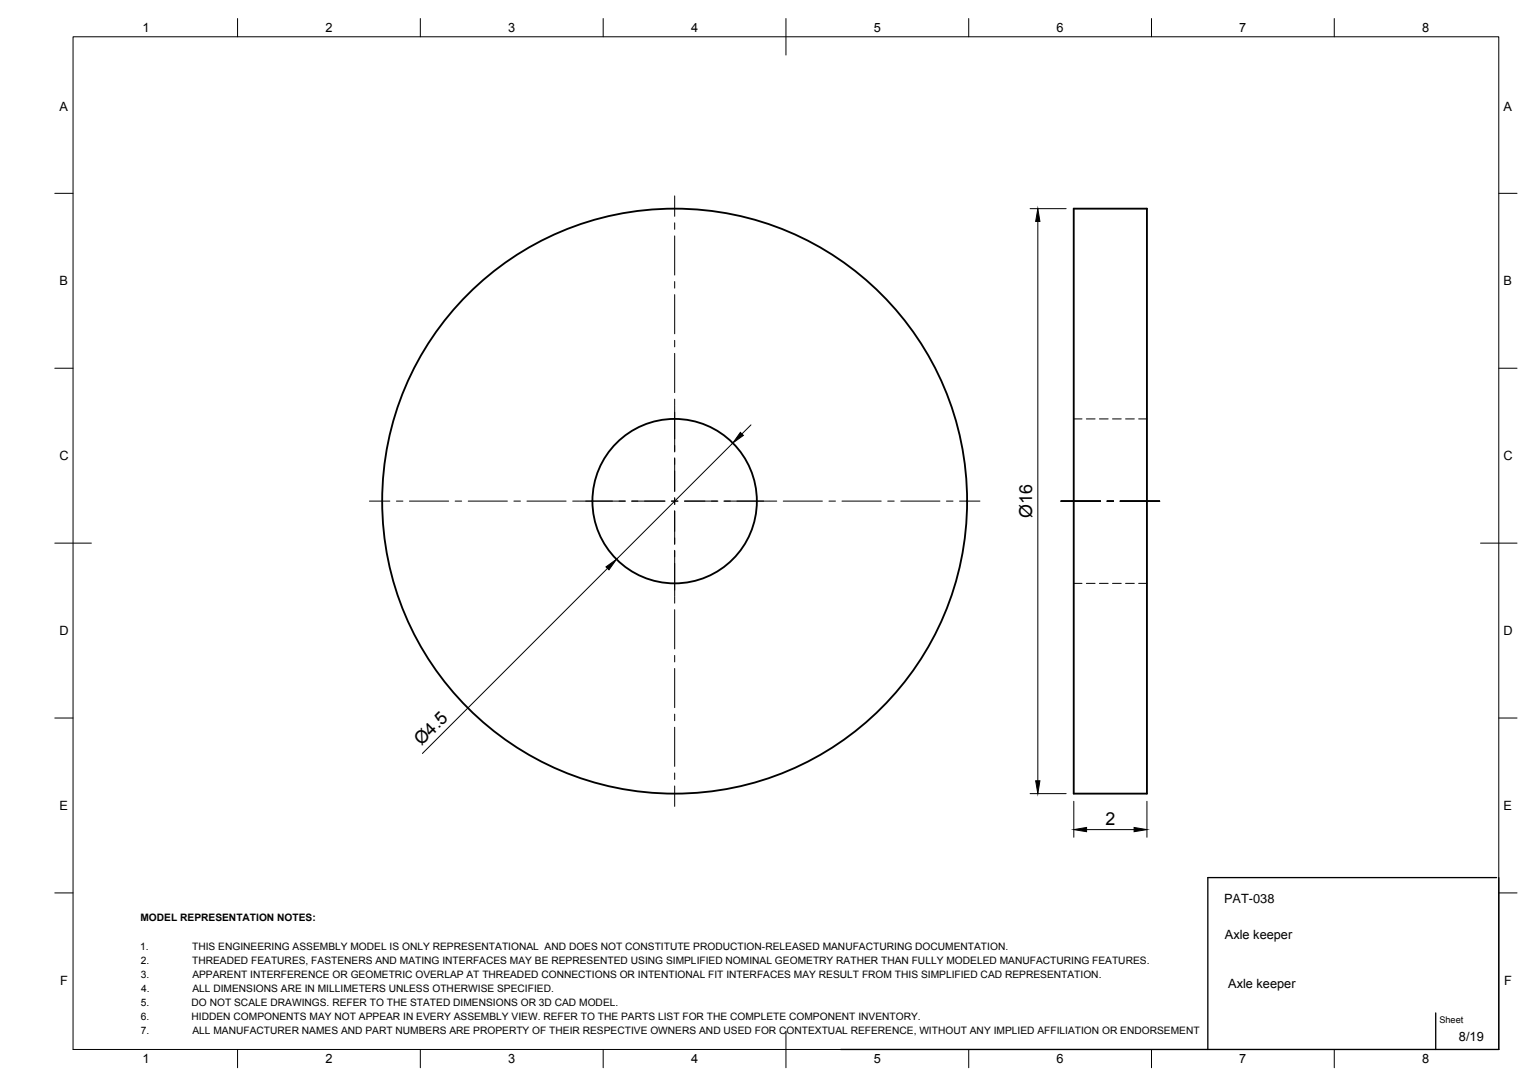
ISO-10303-21;
HEADER;
/* Generated by software containing ST-Developer
 * from STEP Tools, Inc. (www.steptools.com) 
 */

FILE_DESCRIPTION(
/* description */ ('Fork-mounted skate wheel'),
/* implementation_level */ '2;1');

FILE_NAME(
/* name */ 'Axle keeper.step',
/* time_stamp */ '2026-10-29T16:11:26-07:00',
/* author */ (''),
/* organization */ (''),
/* preprocessor_version */ 'ST-DEVELOPER v20.2',
/* originating_system */ 'Autodesk Translation Framework v15.17.0.0',
/* authorisation */ '');

FILE_SCHEMA (('AUTOMOTIVE_DESIGN { 1 0 10303 214 3 1 1 }'));
ENDSEC;

DATA;
#10=MECHANICAL_DESIGN_GEOMETRIC_PRESENTATION_REPRESENTATION('',(#149),#3688);
#125=SHAPE_REPRESENTATION_RELATIONSHIP('SRR','None',#3748,#137);
#137=ADVANCED_BREP_SHAPE_REPRESENTATION('',(#168),#3677);
#149=STYLED_ITEM('',(#3896),#168);
#168=MANIFOLD_SOLID_BREP('Body1',#1810);
#201=FACE_BOUND('',#443,.T.);
#202=FACE_BOUND('',#445,.T.);
#241=PLANE('',#2027);
#242=PLANE('',#2028);
#309=FACE_OUTER_BOUND('',#440,.T.);
#310=FACE_OUTER_BOUND('',#441,.T.);
#311=FACE_OUTER_BOUND('',#442,.T.);
#312=FACE_OUTER_BOUND('',#444,.T.);
#440=EDGE_LOOP('',(#1355,#1356,#1357,#1358));
#441=EDGE_LOOP('',(#1359,#1360,#1361,#1362));
#442=EDGE_LOOP('',(#1363));
#443=EDGE_LOOP('',(#1364));
#444=EDGE_LOOP('',(#1365));
#445=EDGE_LOOP('',(#1366));
#585=LINE('',#2995,#679);
#586=LINE('',#3001,#680);
#679=VECTOR('',#2394,0.225);
#680=VECTOR('',#2401,0.8);
#748=CIRCLE('',#2022,0.225);
#749=CIRCLE('',#2023,0.225);
#750=CIRCLE('',#2025,0.8);
#751=CIRCLE('',#2026,0.8);
#886=VERTEX_POINT('',#2992);
#887=VERTEX_POINT('',#2994);
#888=VERTEX_POINT('',#2998);
#889=VERTEX_POINT('',#3000);
#1064=EDGE_CURVE('',#886,#886,#748,.T.);
#1065=EDGE_CURVE('',#886,#887,#585,.T.);
#1066=EDGE_CURVE('',#887,#887,#749,.T.);
#1067=EDGE_CURVE('',#888,#888,#750,.T.);
#1068=EDGE_CURVE('',#888,#889,#586,.T.);
#1069=EDGE_CURVE('',#889,#889,#751,.T.);
#1355=ORIENTED_EDGE('',*,*,#1064,.F.);
#1356=ORIENTED_EDGE('',*,*,#1065,.T.);
#1357=ORIENTED_EDGE('',*,*,#1066,.T.);
#1358=ORIENTED_EDGE('',*,*,#1065,.F.);
#1359=ORIENTED_EDGE('',*,*,#1067,.F.);
#1360=ORIENTED_EDGE('',*,*,#1068,.T.);
#1361=ORIENTED_EDGE('',*,*,#1069,.T.);
#1362=ORIENTED_EDGE('',*,*,#1068,.F.);
#1363=ORIENTED_EDGE('',*,*,#1067,.T.);
#1364=ORIENTED_EDGE('',*,*,#1064,.T.);
#1365=ORIENTED_EDGE('',*,*,#1069,.F.);
#1366=ORIENTED_EDGE('',*,*,#1066,.F.);
#1672=CYLINDRICAL_SURFACE('',#2021,0.225);
#1673=CYLINDRICAL_SURFACE('',#2024,0.8);
#1727=ADVANCED_FACE('',(#309),#1672,.F.);
#1728=ADVANCED_FACE('',(#310),#1673,.T.);
#1729=ADVANCED_FACE('',(#311,#201),#241,.T.);
#1730=ADVANCED_FACE('',(#312,#202),#242,.F.);
#1810=CLOSED_SHELL('',(#1727,#1728,#1729,#1730));
#2020=AXIS2_PLACEMENT_3D('',#2990,#2388,#2389);
#2021=AXIS2_PLACEMENT_3D('',#2991,#2390,#2391);
#2022=AXIS2_PLACEMENT_3D('',#2993,#2392,#2393);
#2023=AXIS2_PLACEMENT_3D('',#2996,#2395,#2396);
#2024=AXIS2_PLACEMENT_3D('',#2997,#2397,#2398);
#2025=AXIS2_PLACEMENT_3D('',#2999,#2399,#2400);
#2026=AXIS2_PLACEMENT_3D('',#3002,#2402,#2403);
#2027=AXIS2_PLACEMENT_3D('',#3003,#2404,#2405);
#2028=AXIS2_PLACEMENT_3D('',#3004,#2406,#2407);
#2388=DIRECTION('axis',(0.,0.,1.));
#2389=DIRECTION('refdir',(1.,0.,0.));
#2390=DIRECTION('center_axis',(0.,1.,0.));
#2391=DIRECTION('ref_axis',(1.,0.,0.));
#2392=DIRECTION('center_axis',(0.,-1.,0.));
#2393=DIRECTION('ref_axis',(1.,0.,0.));
#2394=DIRECTION('',(0.,-1.,0.));
#2395=DIRECTION('center_axis',(0.,-1.,0.));
#2396=DIRECTION('ref_axis',(1.,0.,0.));
#2397=DIRECTION('center_axis',(0.,1.,0.));
#2398=DIRECTION('ref_axis',(1.,0.,0.));
#2399=DIRECTION('center_axis',(0.,1.,0.));
#2400=DIRECTION('ref_axis',(1.,0.,0.));
#2401=DIRECTION('',(0.,-1.,0.));
#2402=DIRECTION('center_axis',(0.,1.,0.));
#2403=DIRECTION('ref_axis',(1.,0.,0.));
#2404=DIRECTION('center_axis',(0.,1.,0.));
#2405=DIRECTION('ref_axis',(1.,0.,0.));
#2406=DIRECTION('center_axis',(0.,1.,0.));
#2407=DIRECTION('ref_axis',(1.,0.,0.));
#2990=CARTESIAN_POINT('',(0.,0.,0.));
#2991=CARTESIAN_POINT('Origin',(0.,2.2,4.));
#2992=CARTESIAN_POINT('',(-0.225,2.4,4.));
#2993=CARTESIAN_POINT('Origin',(0.,2.4,4.));
#2994=CARTESIAN_POINT('',(-0.225,2.2,4.));
#2995=CARTESIAN_POINT('',(-0.225,2.2,4.));
#2996=CARTESIAN_POINT('Origin',(0.,2.2,4.));
#2997=CARTESIAN_POINT('Origin',(0.,2.2,4.));
#2998=CARTESIAN_POINT('',(-0.8,2.4,4.));
#2999=CARTESIAN_POINT('Origin',(0.,2.4,4.));
#3000=CARTESIAN_POINT('',(-0.8,2.2,4.));
#3001=CARTESIAN_POINT('',(-0.8,2.2,4.));
#3002=CARTESIAN_POINT('Origin',(0.,2.2,4.));
#3003=CARTESIAN_POINT('Origin',(0.,2.4,4.));
#3004=CARTESIAN_POINT('Origin',(0.,2.2,4.));
#3660=UNCERTAINTY_MEASURE_WITH_UNIT(LENGTH_MEASURE(0.001),#3689,
'DISTANCE_ACCURACY_VALUE',
'Maximum model space distance between geometric entities at asserted c
onnectivities');
#3671=UNCERTAINTY_MEASURE_WITH_UNIT(LENGTH_MEASURE(0.001),#3689,
'DISTANCE_ACCURACY_VALUE',
'Maximum model space distance between geometric entities at asserted c
onnectivities');
#3677=(
GEOMETRIC_REPRESENTATION_CONTEXT(3)
GLOBAL_UNCERTAINTY_ASSIGNED_CONTEXT((#3660))
GLOBAL_UNIT_ASSIGNED_CONTEXT((#3689,#3691,#3692))
REPRESENTATION_CONTEXT('','3D')
);
#3688=(
GEOMETRIC_REPRESENTATION_CONTEXT(3)
GLOBAL_UNCERTAINTY_ASSIGNED_CONTEXT((#3671))
GLOBAL_UNIT_ASSIGNED_CONTEXT((#3689,#3691,#3692))
REPRESENTATION_CONTEXT('','3D')
);
#3689=(
LENGTH_UNIT()
NAMED_UNIT(*)
SI_UNIT(.CENTI.,.METRE.)
);
#3691=(
NAMED_UNIT(*)
PLANE_ANGLE_UNIT()
SI_UNIT($,.RADIAN.)
);
#3692=(
NAMED_UNIT(*)
SI_UNIT($,.STERADIAN.)
SOLID_ANGLE_UNIT()
);
#3698=SHAPE_DEFINITION_REPRESENTATION(#3714,#3748);
#3714=PRODUCT_DEFINITION_SHAPE('',$,#3765);
#3748=SHAPE_REPRESENTATION('',(#2020),#3677);
#3759=PRODUCT_DEFINITION_CONTEXT('part definition',#3809,'design');
#3765=PRODUCT_DEFINITION('Axle keeper','Axle keeper',#3781,#3759);
#3781=PRODUCT_DEFINITION_FORMATION('',$,#3816);
#3809=APPLICATION_CONTEXT(
'Core Data for Automotive Mechanical Design Process');
#3810=PRODUCT_CONTEXT('part definition',#3809,'mechanical');
#3816=PRODUCT('Axle keeper','Axle keeper','Axle keeper',(#3810));
#3890=COLOUR_RGB('Grey',0.48,0.52,0.57);
#3891=FILL_AREA_STYLE_COLOUR('',#3890);
#3892=FILL_AREA_STYLE('',(#3891));
#3893=SURFACE_STYLE_FILL_AREA(#3892);
#3894=SURFACE_SIDE_STYLE('',(#3893));
#3895=SURFACE_STYLE_USAGE(.BOTH.,#3894);
#3896=PRESENTATION_STYLE_ASSIGNMENT((#3895));
ENDSEC;
END-ISO-10303-21;
